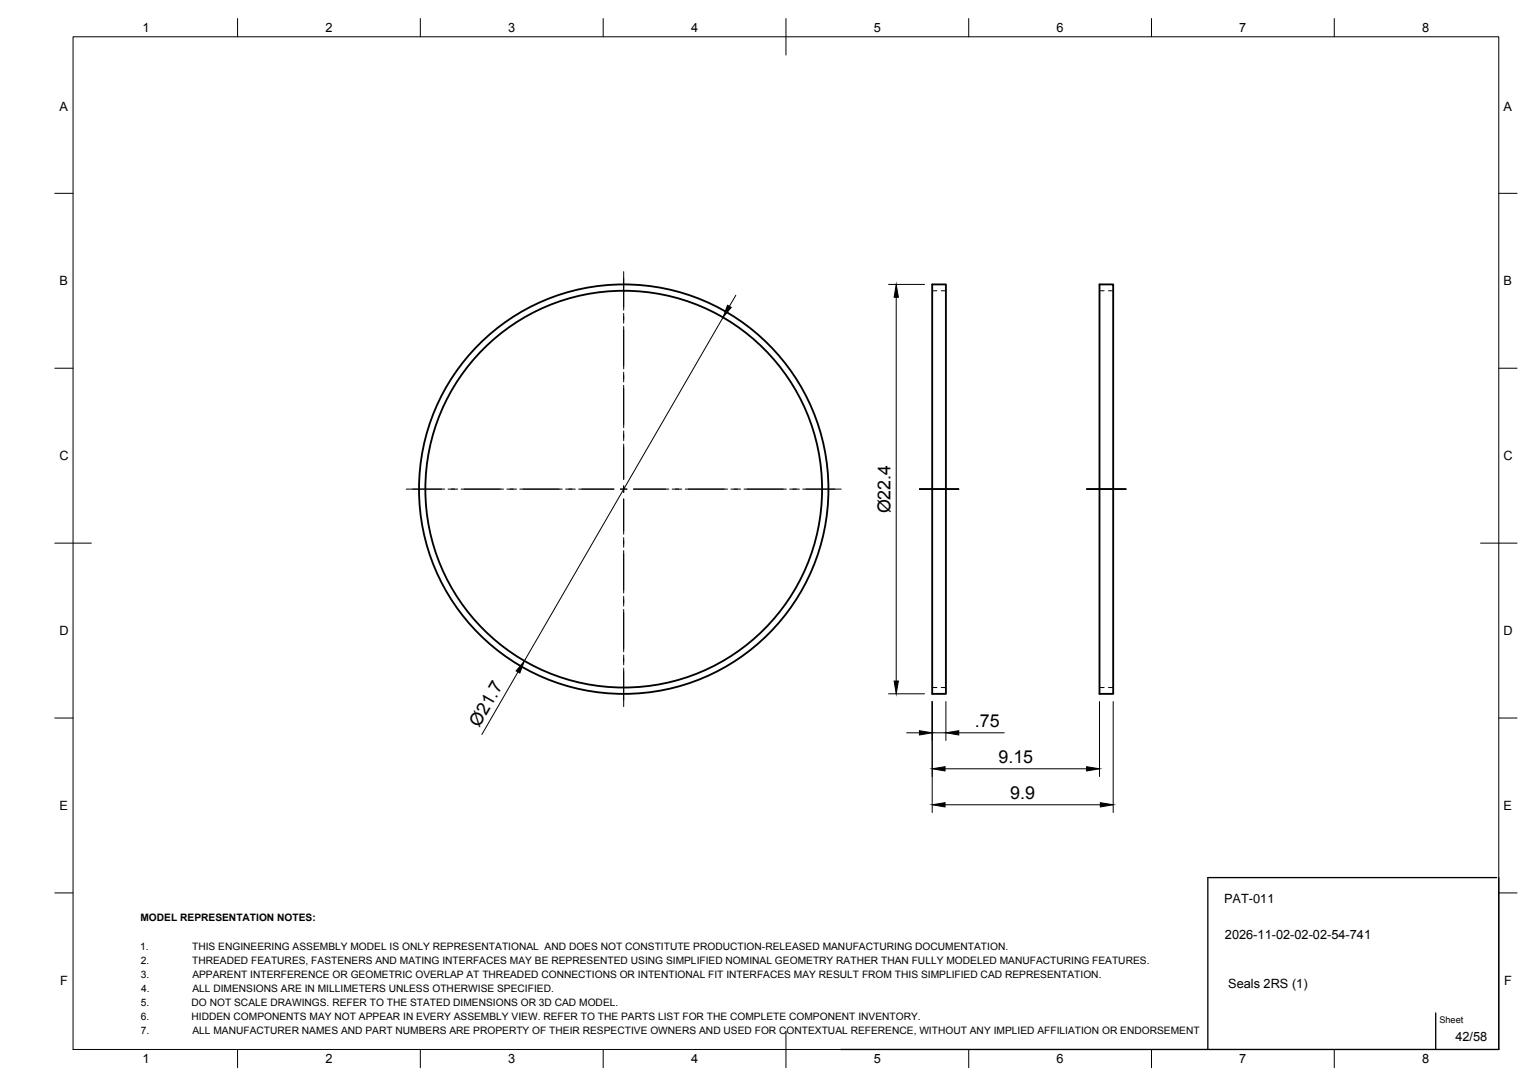
ISO-10303-21;
HEADER;
/* Generated by software containing ST-Developer
 * from STEP Tools, Inc. (www.steptools.com) 
 */

FILE_DESCRIPTION(
/* description */ ('Belt tension measurement rig'),
/* implementation_level */ '2;1');

FILE_NAME(
/* name */ 'Seals 2RS (1).step',
/* time_stamp */ '2026-10-28T03:24:44-07:00',
/* author */ (''),
/* organization */ (''),
/* preprocessor_version */ 'ST-DEVELOPER v20.2',
/* originating_system */ 'Autodesk Translation Framework v15.17.0.0',
/* authorisation */ '');

FILE_SCHEMA (('AUTOMOTIVE_DESIGN { 1 0 10303 214 3 1 1 }'));
ENDSEC;

DATA;
#10=MECHANICAL_DESIGN_GEOMETRIC_PRESENTATION_REPRESENTATION('',(#741,#742),#23587);
#617=SHAPE_REPRESENTATION_RELATIONSHIP('SRR','None',#23866,#672);
#672=ADVANCED_BREP_SHAPE_REPRESENTATION('',(#810,#811),#23564);
#741=STYLED_ITEM('',(#24211),#810);
#742=STYLED_ITEM('',(#24211),#811);
#810=MANIFOLD_SOLID_BREP('Body1',#12247);
#811=MANIFOLD_SOLID_BREP('Body2',#12248);
#979=FACE_BOUND('',#2630,.T.);
#980=FACE_BOUND('',#2633,.T.);
#981=FACE_BOUND('',#2636,.T.);
#982=FACE_BOUND('',#2639,.T.);
#1262=PLANE('',#13760);
#1263=PLANE('',#13765);
#1264=PLANE('',#13768);
#1265=PLANE('',#13773);
#1775=FACE_OUTER_BOUND('',#2629,.T.);
#1776=FACE_OUTER_BOUND('',#2631,.T.);
#1777=FACE_OUTER_BOUND('',#2632,.T.);
#1778=FACE_OUTER_BOUND('',#2634,.T.);
#1779=FACE_OUTER_BOUND('',#2635,.T.);
#1780=FACE_OUTER_BOUND('',#2637,.T.);
#1781=FACE_OUTER_BOUND('',#2638,.T.);
#1782=FACE_OUTER_BOUND('',#2640,.T.);
#2629=EDGE_LOOP('',(#9836));
#2630=EDGE_LOOP('',(#9837));
#2631=EDGE_LOOP('',(#9838,#9839,#9840,#9841));
#2632=EDGE_LOOP('',(#9842));
#2633=EDGE_LOOP('',(#9843));
#2634=EDGE_LOOP('',(#9844,#9845,#9846,#9847));
#2635=EDGE_LOOP('',(#9848));
#2636=EDGE_LOOP('',(#9849));
#2637=EDGE_LOOP('',(#9850,#9851,#9852,#9853));
#2638=EDGE_LOOP('',(#9854));
#2639=EDGE_LOOP('',(#9855));
#2640=EDGE_LOOP('',(#9856,#9857,#9858,#9859));
#3466=LINE('',#21350,#4217);
#3467=LINE('',#21355,#4218);
#3468=LINE('',#21364,#4219);
#3469=LINE('',#21369,#4220);
#4217=VECTOR('',#16793,1.119765);
#4218=VECTOR('',#16800,1.085235);
#4219=VECTOR('',#16811,1.119765);
#4220=VECTOR('',#16818,1.085235);
#4881=CIRCLE('',#13761,1.119765);
#4882=CIRCLE('',#13762,1.085235);
#4883=CIRCLE('',#13764,1.119765);
#4884=CIRCLE('',#13766,1.085235);
#4885=CIRCLE('',#13769,1.119765);
#4886=CIRCLE('',#13770,1.085235);
#4887=CIRCLE('',#13772,1.119765);
#4888=CIRCLE('',#13774,1.085235);
#5884=VERTEX_POINT('',#21343);
#5885=VERTEX_POINT('',#21345);
#5886=VERTEX_POINT('',#21348);
#5887=VERTEX_POINT('',#21352);
#5888=VERTEX_POINT('',#21357);
#5889=VERTEX_POINT('',#21359);
#5890=VERTEX_POINT('',#21362);
#5891=VERTEX_POINT('',#21366);
#7277=EDGE_CURVE('',#5884,#5884,#4881,.T.);
#7278=EDGE_CURVE('',#5885,#5885,#4882,.T.);
#7279=EDGE_CURVE('',#5886,#5886,#4883,.T.);
#7280=EDGE_CURVE('',#5886,#5884,#3466,.T.);
#7281=EDGE_CURVE('',#5887,#5887,#4884,.T.);
#7282=EDGE_CURVE('',#5887,#5885,#3467,.T.);
#7283=EDGE_CURVE('',#5888,#5888,#4885,.T.);
#7284=EDGE_CURVE('',#5889,#5889,#4886,.T.);
#7285=EDGE_CURVE('',#5890,#5890,#4887,.T.);
#7286=EDGE_CURVE('',#5890,#5888,#3468,.T.);
#7287=EDGE_CURVE('',#5891,#5891,#4888,.T.);
#7288=EDGE_CURVE('',#5891,#5889,#3469,.T.);
#9836=ORIENTED_EDGE('',*,*,#7277,.F.);
#9837=ORIENTED_EDGE('',*,*,#7278,.T.);
#9838=ORIENTED_EDGE('',*,*,#7279,.F.);
#9839=ORIENTED_EDGE('',*,*,#7280,.T.);
#9840=ORIENTED_EDGE('',*,*,#7277,.T.);
#9841=ORIENTED_EDGE('',*,*,#7280,.F.);
#9842=ORIENTED_EDGE('',*,*,#7279,.T.);
#9843=ORIENTED_EDGE('',*,*,#7281,.F.);
#9844=ORIENTED_EDGE('',*,*,#7281,.T.);
#9845=ORIENTED_EDGE('',*,*,#7282,.T.);
#9846=ORIENTED_EDGE('',*,*,#7278,.F.);
#9847=ORIENTED_EDGE('',*,*,#7282,.F.);
#9848=ORIENTED_EDGE('',*,*,#7283,.F.);
#9849=ORIENTED_EDGE('',*,*,#7284,.T.);
#9850=ORIENTED_EDGE('',*,*,#7285,.F.);
#9851=ORIENTED_EDGE('',*,*,#7286,.T.);
#9852=ORIENTED_EDGE('',*,*,#7283,.T.);
#9853=ORIENTED_EDGE('',*,*,#7286,.F.);
#9854=ORIENTED_EDGE('',*,*,#7285,.T.);
#9855=ORIENTED_EDGE('',*,*,#7287,.F.);
#9856=ORIENTED_EDGE('',*,*,#7287,.T.);
#9857=ORIENTED_EDGE('',*,*,#7288,.T.);
#9858=ORIENTED_EDGE('',*,*,#7284,.F.);
#9859=ORIENTED_EDGE('',*,*,#7288,.F.);
#11311=CYLINDRICAL_SURFACE('',#13763,1.119765);
#11312=CYLINDRICAL_SURFACE('',#13767,1.085235);
#11313=CYLINDRICAL_SURFACE('',#13771,1.119765);
#11314=CYLINDRICAL_SURFACE('',#13775,1.085235);
#11916=ADVANCED_FACE('',(#1775,#979),#1262,.T.);
#11917=ADVANCED_FACE('',(#1776),#11311,.T.);
#11918=ADVANCED_FACE('',(#1777,#980),#1263,.T.);
#11919=ADVANCED_FACE('',(#1778),#11312,.F.);
#11920=ADVANCED_FACE('',(#1779,#981),#1264,.T.);
#11921=ADVANCED_FACE('',(#1780),#11313,.T.);
#11922=ADVANCED_FACE('',(#1781,#982),#1265,.T.);
#11923=ADVANCED_FACE('',(#1782),#11314,.F.);
#12247=CLOSED_SHELL('',(#11916,#11917,#11918,#11919));
#12248=CLOSED_SHELL('',(#11920,#11921,#11922,#11923));
#13759=AXIS2_PLACEMENT_3D('',#21341,#16781,#16782);
#13760=AXIS2_PLACEMENT_3D('',#21342,#16783,#16784);
#13761=AXIS2_PLACEMENT_3D('',#21344,#16785,#16786);
#13762=AXIS2_PLACEMENT_3D('',#21346,#16787,#16788);
#13763=AXIS2_PLACEMENT_3D('',#21347,#16789,#16790);
#13764=AXIS2_PLACEMENT_3D('',#21349,#16791,#16792);
#13765=AXIS2_PLACEMENT_3D('',#21351,#16794,#16795);
#13766=AXIS2_PLACEMENT_3D('',#21353,#16796,#16797);
#13767=AXIS2_PLACEMENT_3D('',#21354,#16798,#16799);
#13768=AXIS2_PLACEMENT_3D('',#21356,#16801,#16802);
#13769=AXIS2_PLACEMENT_3D('',#21358,#16803,#16804);
#13770=AXIS2_PLACEMENT_3D('',#21360,#16805,#16806);
#13771=AXIS2_PLACEMENT_3D('',#21361,#16807,#16808);
#13772=AXIS2_PLACEMENT_3D('',#21363,#16809,#16810);
#13773=AXIS2_PLACEMENT_3D('',#21365,#16812,#16813);
#13774=AXIS2_PLACEMENT_3D('',#21367,#16814,#16815);
#13775=AXIS2_PLACEMENT_3D('',#21368,#16816,#16817);
#16781=DIRECTION('axis',(0.,0.,1.));
#16782=DIRECTION('refdir',(1.,0.,0.));
#16783=DIRECTION('center_axis',(0.,1.,0.));
#16784=DIRECTION('ref_axis',(0.,0.,1.));
#16785=DIRECTION('center_axis',(0.,-1.,0.));
#16786=DIRECTION('ref_axis',(1.,0.,0.));
#16787=DIRECTION('center_axis',(0.,-1.,0.));
#16788=DIRECTION('ref_axis',(1.,0.,0.));
#16789=DIRECTION('center_axis',(0.,-1.,0.));
#16790=DIRECTION('ref_axis',(1.,0.,0.));
#16791=DIRECTION('center_axis',(0.,-1.,0.));
#16792=DIRECTION('ref_axis',(1.,0.,0.));
#16793=DIRECTION('',(0.,1.,0.));
#16794=DIRECTION('center_axis',(0.,-1.,0.));
#16795=DIRECTION('ref_axis',(0.,0.,-1.));
#16796=DIRECTION('center_axis',(0.,-1.,0.));
#16797=DIRECTION('ref_axis',(1.,0.,0.));
#16798=DIRECTION('center_axis',(0.,-1.,0.));
#16799=DIRECTION('ref_axis',(1.,0.,0.));
#16800=DIRECTION('',(0.,1.,0.));
#16801=DIRECTION('center_axis',(0.,1.,0.));
#16802=DIRECTION('ref_axis',(0.,0.,1.));
#16803=DIRECTION('center_axis',(0.,-1.,0.));
#16804=DIRECTION('ref_axis',(1.,0.,0.));
#16805=DIRECTION('center_axis',(0.,-1.,0.));
#16806=DIRECTION('ref_axis',(1.,0.,0.));
#16807=DIRECTION('center_axis',(0.,-1.,0.));
#16808=DIRECTION('ref_axis',(1.,0.,0.));
#16809=DIRECTION('center_axis',(0.,-1.,0.));
#16810=DIRECTION('ref_axis',(1.,0.,0.));
#16811=DIRECTION('',(0.,1.,0.));
#16812=DIRECTION('center_axis',(0.,-1.,0.));
#16813=DIRECTION('ref_axis',(0.,0.,-1.));
#16814=DIRECTION('center_axis',(0.,-1.,0.));
#16815=DIRECTION('ref_axis',(1.,0.,0.));
#16816=DIRECTION('center_axis',(0.,-1.,0.));
#16817=DIRECTION('ref_axis',(1.,0.,0.));
#16818=DIRECTION('',(0.,1.,0.));
#21341=CARTESIAN_POINT('',(0.,0.,0.));
#21342=CARTESIAN_POINT('Origin',(1.119765,0.495,0.));
#21343=CARTESIAN_POINT('',(-1.119765,0.495,-1.37131662304724E-16));
#21344=CARTESIAN_POINT('Origin',(0.,0.495,0.));
#21345=CARTESIAN_POINT('',(-1.085235,0.495,-1.32902956907268E-16));
#21346=CARTESIAN_POINT('Origin',(0.,0.495,0.));
#21347=CARTESIAN_POINT('Origin',(0.,0.4575,0.));
#21348=CARTESIAN_POINT('',(-1.119765,0.42,-1.37131662304724E-16));
#21349=CARTESIAN_POINT('Origin',(0.,0.42,0.));
#21350=CARTESIAN_POINT('',(-1.119765,0.4575,-1.37131662304724E-16));
#21351=CARTESIAN_POINT('Origin',(1.085235,0.42,0.));
#21352=CARTESIAN_POINT('',(-1.085235,0.42,-1.32902956907268E-16));
#21353=CARTESIAN_POINT('Origin',(0.,0.42,0.));
#21354=CARTESIAN_POINT('Origin',(0.,0.4575,0.));
#21355=CARTESIAN_POINT('',(-1.085235,0.4575,-1.32902956907268E-16));
#21356=CARTESIAN_POINT('Origin',(1.119765,-0.42,0.));
#21357=CARTESIAN_POINT('',(-1.119765,-0.42,-1.37131662304724E-16));
#21358=CARTESIAN_POINT('Origin',(0.,-0.42,0.));
#21359=CARTESIAN_POINT('',(-1.085235,-0.42,-1.32902956907268E-16));
#21360=CARTESIAN_POINT('Origin',(0.,-0.42,0.));
#21361=CARTESIAN_POINT('Origin',(0.,-0.4575,0.));
#21362=CARTESIAN_POINT('',(-1.119765,-0.495,-1.37131662304724E-16));
#21363=CARTESIAN_POINT('Origin',(0.,-0.495,0.));
#21364=CARTESIAN_POINT('',(-1.119765,-0.4575,-1.37131662304724E-16));
#21365=CARTESIAN_POINT('Origin',(1.085235,-0.495,0.));
#21366=CARTESIAN_POINT('',(-1.085235,-0.495,-1.32902956907268E-16));
#21367=CARTESIAN_POINT('Origin',(0.,-0.495,0.));
#21368=CARTESIAN_POINT('Origin',(0.,-0.4575,0.));
#21369=CARTESIAN_POINT('',(-1.085235,-0.4575,-1.32902956907268E-16));
#23499=UNCERTAINTY_MEASURE_WITH_UNIT(LENGTH_MEASURE(0.001),#23588,
'DISTANCE_ACCURACY_VALUE',
'Maximum model space distance between geometric entities at asserted c
onnectivities');
#23522=UNCERTAINTY_MEASURE_WITH_UNIT(LENGTH_MEASURE(0.001),#23588,
'DISTANCE_ACCURACY_VALUE',
'Maximum model space distance between geometric entities at asserted c
onnectivities');
#23564=(
GEOMETRIC_REPRESENTATION_CONTEXT(3)
GLOBAL_UNCERTAINTY_ASSIGNED_CONTEXT((#23499))
GLOBAL_UNIT_ASSIGNED_CONTEXT((#23588,#23590,#23591))
REPRESENTATION_CONTEXT('','3D')
);
#23587=(
GEOMETRIC_REPRESENTATION_CONTEXT(3)
GLOBAL_UNCERTAINTY_ASSIGNED_CONTEXT((#23522))
GLOBAL_UNIT_ASSIGNED_CONTEXT((#23588,#23590,#23591))
REPRESENTATION_CONTEXT('','3D')
);
#23588=(
LENGTH_UNIT()
NAMED_UNIT(*)
SI_UNIT(.CENTI.,.METRE.)
);
#23590=(
NAMED_UNIT(*)
PLANE_ANGLE_UNIT()
SI_UNIT($,.RADIAN.)
);
#23591=(
NAMED_UNIT(*)
SI_UNIT($,.STERADIAN.)
SOLID_ANGLE_UNIT()
);
#23633=SHAPE_DEFINITION_REPRESENTATION(#23705,#23866);
#23705=PRODUCT_DEFINITION_SHAPE('',$,#23931);
#23866=SHAPE_REPRESENTATION('',(#13759),#23564);
#23889=PRODUCT_DEFINITION_CONTEXT('part definition',#24083,'design');
#23931=PRODUCT_DEFINITION('Seals 2RS (1)','Seals 2RS (1)',#23995,#23889);
#23995=PRODUCT_DEFINITION_FORMATION('',$,#24126);
#24083=APPLICATION_CONTEXT(
'Core Data for Automotive Mechanical Design Process');
#24084=PRODUCT_CONTEXT('part definition',#24083,'mechanical');
#24126=PRODUCT('Seals 2RS (1)','Seals 2RS (1)','Seals 2RS (1)',(#24084));
#24205=COLOUR_RGB('Grey',0.48,0.52,0.57);
#24206=FILL_AREA_STYLE_COLOUR('',#24205);
#24207=FILL_AREA_STYLE('',(#24206));
#24208=SURFACE_STYLE_FILL_AREA(#24207);
#24209=SURFACE_SIDE_STYLE('',(#24208));
#24210=SURFACE_STYLE_USAGE(.BOTH.,#24209);
#24211=PRESENTATION_STYLE_ASSIGNMENT((#24210));
ENDSEC;
END-ISO-10303-21;
